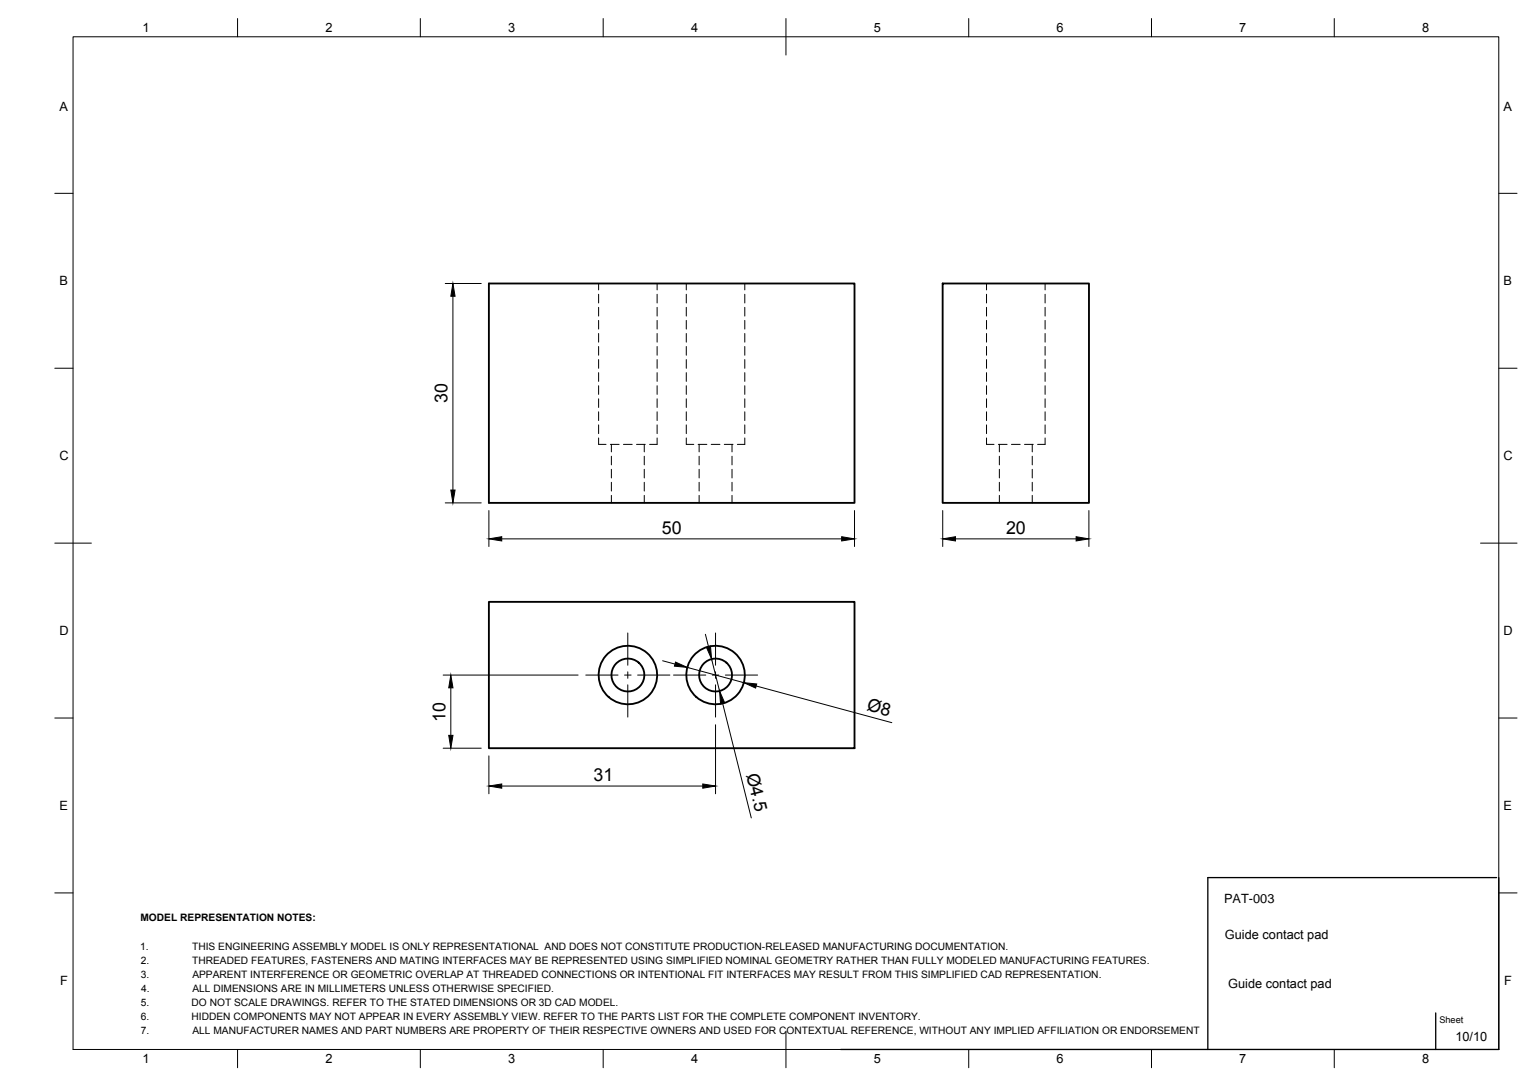
ISO-10303-21;
HEADER;
/* Generated by software containing ST-Developer
 * from STEP Tools, Inc. (www.steptools.com) 
 */

FILE_DESCRIPTION(
/* description */ ('PAT-003'),
/* implementation_level */ '2;1');

FILE_NAME(
/* name */ 'Guide contact pad.step',
/* time_stamp */ '2026-10-29T15:45:40-07:00',
/* author */ (''),
/* organization */ (''),
/* preprocessor_version */ 'ST-DEVELOPER v20.2',
/* originating_system */ 'Autodesk Translation Framework v15.17.0.0',
/* authorisation */ '');

FILE_SCHEMA (('AUTOMOTIVE_DESIGN { 1 0 10303 214 3 1 1 }'));
ENDSEC;

DATA;
#10=MECHANICAL_DESIGN_GEOMETRIC_PRESENTATION_REPRESENTATION('',(#154),#5761);
#130=SHAPE_REPRESENTATION_RELATIONSHIP('SRR','None',#5825,#142);
#142=ADVANCED_BREP_SHAPE_REPRESENTATION('',(#165),#5756);
#154=STYLED_ITEM('',(#5942),#165);
#165=MANIFOLD_SOLID_BREP('Body1',#3329);
#192=FACE_BOUND('',#674,.T.);
#193=FACE_BOUND('',#677,.T.);
#194=FACE_BOUND('',#685,.T.);
#195=FACE_BOUND('',#686,.T.);
#196=FACE_BOUND('',#688,.T.);
#197=FACE_BOUND('',#689,.T.);
#303=PLANE('',#3651);
#304=PLANE('',#3656);
#305=PLANE('',#3662);
#306=PLANE('',#3663);
#307=PLANE('',#3664);
#308=PLANE('',#3665);
#309=PLANE('',#3666);
#310=PLANE('',#3667);
#462=FACE_OUTER_BOUND('',#672,.T.);
#463=FACE_OUTER_BOUND('',#673,.T.);
#464=FACE_OUTER_BOUND('',#675,.T.);
#465=FACE_OUTER_BOUND('',#676,.T.);
#466=FACE_OUTER_BOUND('',#678,.T.);
#467=FACE_OUTER_BOUND('',#679,.T.);
#468=FACE_OUTER_BOUND('',#680,.T.);
#469=FACE_OUTER_BOUND('',#681,.T.);
#470=FACE_OUTER_BOUND('',#682,.T.);
#471=FACE_OUTER_BOUND('',#683,.T.);
#472=FACE_OUTER_BOUND('',#684,.T.);
#473=FACE_OUTER_BOUND('',#687,.T.);
#672=EDGE_LOOP('',(#2806,#2807,#2808,#2809));
#673=EDGE_LOOP('',(#2810));
#674=EDGE_LOOP('',(#2811));
#675=EDGE_LOOP('',(#2812,#2813,#2814,#2815));
#676=EDGE_LOOP('',(#2816));
#677=EDGE_LOOP('',(#2817));
#678=EDGE_LOOP('',(#2818,#2819,#2820,#2821));
#679=EDGE_LOOP('',(#2822,#2823,#2824,#2825));
#680=EDGE_LOOP('',(#2826,#2827,#2828,#2829));
#681=EDGE_LOOP('',(#2830,#2831,#2832,#2833));
#682=EDGE_LOOP('',(#2834,#2835,#2836,#2837));
#683=EDGE_LOOP('',(#2838,#2839,#2840,#2841));
#684=EDGE_LOOP('',(#2842,#2843,#2844,#2845));
#685=EDGE_LOOP('',(#2846));
#686=EDGE_LOOP('',(#2847));
#687=EDGE_LOOP('',(#2848,#2849,#2850,#2851));
#688=EDGE_LOOP('',(#2852));
#689=EDGE_LOOP('',(#2853));
#992=LINE('',#5383,#1314);
#993=LINE('',#5392,#1315);
#994=LINE('',#5400,#1316);
#995=LINE('',#5404,#1317);
#996=LINE('',#5408,#1318);
#997=LINE('',#5410,#1319);
#998=LINE('',#5412,#1320);
#999=LINE('',#5413,#1321);
#1000=LINE('',#5416,#1322);
#1001=LINE('',#5418,#1323);
#1002=LINE('',#5419,#1324);
#1003=LINE('',#5422,#1325);
#1004=LINE('',#5424,#1326);
#1005=LINE('',#5425,#1327);
#1006=LINE('',#5427,#1328);
#1007=LINE('',#5428,#1329);
#1314=VECTOR('',#4391,0.4);
#1315=VECTOR('',#4402,0.4);
#1316=VECTOR('',#4413,0.225);
#1317=VECTOR('',#4418,0.225);
#1318=VECTOR('',#4421,1.);
#1319=VECTOR('',#4422,1.);
#1320=VECTOR('',#4423,1.);
#1321=VECTOR('',#4424,1.);
#1322=VECTOR('',#4427,1.);
#1323=VECTOR('',#4428,1.);
#1324=VECTOR('',#4429,1.);
#1325=VECTOR('',#4432,1.);
#1326=VECTOR('',#4433,1.);
#1327=VECTOR('',#4434,1.);
#1328=VECTOR('',#4437,1.);
#1329=VECTOR('',#4438,1.);
#1442=CIRCLE('',#3649,0.4);
#1443=CIRCLE('',#3650,0.4);
#1444=CIRCLE('',#3652,0.225);
#1445=CIRCLE('',#3654,0.4);
#1446=CIRCLE('',#3655,0.4);
#1447=CIRCLE('',#3657,0.225);
#1448=CIRCLE('',#3659,0.225);
#1449=CIRCLE('',#3661,0.225);
#1686=VERTEX_POINT('',#5380);
#1687=VERTEX_POINT('',#5382);
#1688=VERTEX_POINT('',#5386);
#1689=VERTEX_POINT('',#5389);
#1690=VERTEX_POINT('',#5391);
#1691=VERTEX_POINT('',#5395);
#1692=VERTEX_POINT('',#5398);
#1693=VERTEX_POINT('',#5402);
#1694=VERTEX_POINT('',#5406);
#1695=VERTEX_POINT('',#5407);
#1696=VERTEX_POINT('',#5409);
#1697=VERTEX_POINT('',#5411);
#1698=VERTEX_POINT('',#5415);
#1699=VERTEX_POINT('',#5417);
#1700=VERTEX_POINT('',#5421);
#1701=VERTEX_POINT('',#5423);
#2074=EDGE_CURVE('',#1686,#1686,#1442,.T.);
#2075=EDGE_CURVE('',#1686,#1687,#992,.T.);
#2076=EDGE_CURVE('',#1687,#1687,#1443,.T.);
#2077=EDGE_CURVE('',#1688,#1688,#1444,.T.);
#2078=EDGE_CURVE('',#1689,#1689,#1445,.T.);
#2079=EDGE_CURVE('',#1689,#1690,#993,.T.);
#2080=EDGE_CURVE('',#1690,#1690,#1446,.T.);
#2081=EDGE_CURVE('',#1691,#1691,#1447,.T.);
#2082=EDGE_CURVE('',#1692,#1692,#1448,.T.);
#2083=EDGE_CURVE('',#1692,#1688,#994,.T.);
#2084=EDGE_CURVE('',#1693,#1693,#1449,.T.);
#2085=EDGE_CURVE('',#1693,#1691,#995,.T.);
#2086=EDGE_CURVE('',#1694,#1695,#996,.T.);
#2087=EDGE_CURVE('',#1695,#1696,#997,.T.);
#2088=EDGE_CURVE('',#1697,#1696,#998,.T.);
#2089=EDGE_CURVE('',#1694,#1697,#999,.T.);
#2090=EDGE_CURVE('',#1698,#1694,#1000,.T.);
#2091=EDGE_CURVE('',#1699,#1697,#1001,.T.);
#2092=EDGE_CURVE('',#1698,#1699,#1002,.T.);
#2093=EDGE_CURVE('',#1700,#1698,#1003,.T.);
#2094=EDGE_CURVE('',#1701,#1699,#1004,.T.);
#2095=EDGE_CURVE('',#1700,#1701,#1005,.T.);
#2096=EDGE_CURVE('',#1695,#1700,#1006,.T.);
#2097=EDGE_CURVE('',#1696,#1701,#1007,.T.);
#2806=ORIENTED_EDGE('',*,*,#2074,.F.);
#2807=ORIENTED_EDGE('',*,*,#2075,.T.);
#2808=ORIENTED_EDGE('',*,*,#2076,.F.);
#2809=ORIENTED_EDGE('',*,*,#2075,.F.);
#2810=ORIENTED_EDGE('',*,*,#2074,.T.);
#2811=ORIENTED_EDGE('',*,*,#2077,.F.);
#2812=ORIENTED_EDGE('',*,*,#2078,.F.);
#2813=ORIENTED_EDGE('',*,*,#2079,.T.);
#2814=ORIENTED_EDGE('',*,*,#2080,.F.);
#2815=ORIENTED_EDGE('',*,*,#2079,.F.);
#2816=ORIENTED_EDGE('',*,*,#2078,.T.);
#2817=ORIENTED_EDGE('',*,*,#2081,.F.);
#2818=ORIENTED_EDGE('',*,*,#2082,.F.);
#2819=ORIENTED_EDGE('',*,*,#2083,.T.);
#2820=ORIENTED_EDGE('',*,*,#2077,.T.);
#2821=ORIENTED_EDGE('',*,*,#2083,.F.);
#2822=ORIENTED_EDGE('',*,*,#2084,.F.);
#2823=ORIENTED_EDGE('',*,*,#2085,.T.);
#2824=ORIENTED_EDGE('',*,*,#2081,.T.);
#2825=ORIENTED_EDGE('',*,*,#2085,.F.);
#2826=ORIENTED_EDGE('',*,*,#2086,.T.);
#2827=ORIENTED_EDGE('',*,*,#2087,.T.);
#2828=ORIENTED_EDGE('',*,*,#2088,.F.);
#2829=ORIENTED_EDGE('',*,*,#2089,.F.);
#2830=ORIENTED_EDGE('',*,*,#2090,.T.);
#2831=ORIENTED_EDGE('',*,*,#2089,.T.);
#2832=ORIENTED_EDGE('',*,*,#2091,.F.);
#2833=ORIENTED_EDGE('',*,*,#2092,.F.);
#2834=ORIENTED_EDGE('',*,*,#2093,.T.);
#2835=ORIENTED_EDGE('',*,*,#2092,.T.);
#2836=ORIENTED_EDGE('',*,*,#2094,.F.);
#2837=ORIENTED_EDGE('',*,*,#2095,.F.);
#2838=ORIENTED_EDGE('',*,*,#2096,.T.);
#2839=ORIENTED_EDGE('',*,*,#2095,.T.);
#2840=ORIENTED_EDGE('',*,*,#2097,.F.);
#2841=ORIENTED_EDGE('',*,*,#2087,.F.);
#2842=ORIENTED_EDGE('',*,*,#2097,.T.);
#2843=ORIENTED_EDGE('',*,*,#2094,.T.);
#2844=ORIENTED_EDGE('',*,*,#2091,.T.);
#2845=ORIENTED_EDGE('',*,*,#2088,.T.);
#2846=ORIENTED_EDGE('',*,*,#2076,.T.);
#2847=ORIENTED_EDGE('',*,*,#2080,.T.);
#2848=ORIENTED_EDGE('',*,*,#2096,.F.);
#2849=ORIENTED_EDGE('',*,*,#2086,.F.);
#2850=ORIENTED_EDGE('',*,*,#2090,.F.);
#2851=ORIENTED_EDGE('',*,*,#2093,.F.);
#2852=ORIENTED_EDGE('',*,*,#2082,.T.);
#2853=ORIENTED_EDGE('',*,*,#2084,.T.);
#3112=CYLINDRICAL_SURFACE('',#3648,0.4);
#3113=CYLINDRICAL_SURFACE('',#3653,0.4);
#3114=CYLINDRICAL_SURFACE('',#3658,0.225);
#3115=CYLINDRICAL_SURFACE('',#3660,0.225);
#3255=ADVANCED_FACE('',(#462),#3112,.F.);
#3256=ADVANCED_FACE('',(#463,#192),#303,.T.);
#3257=ADVANCED_FACE('',(#464),#3113,.F.);
#3258=ADVANCED_FACE('',(#465,#193),#304,.T.);
#3259=ADVANCED_FACE('',(#466),#3114,.F.);
#3260=ADVANCED_FACE('',(#467),#3115,.F.);
#3261=ADVANCED_FACE('',(#468),#305,.T.);
#3262=ADVANCED_FACE('',(#469),#306,.T.);
#3263=ADVANCED_FACE('',(#470),#307,.T.);
#3264=ADVANCED_FACE('',(#471),#308,.T.);
#3265=ADVANCED_FACE('',(#472,#194,#195),#309,.T.);
#3266=ADVANCED_FACE('',(#473,#196,#197),#310,.F.);
#3329=CLOSED_SHELL('',(#3255,#3256,#3257,#3258,#3259,#3260,#3261,#3262,
#3263,#3264,#3265,#3266));
#3647=AXIS2_PLACEMENT_3D('',#5378,#4385,#4386);
#3648=AXIS2_PLACEMENT_3D('',#5379,#4387,#4388);
#3649=AXIS2_PLACEMENT_3D('',#5381,#4389,#4390);
#3650=AXIS2_PLACEMENT_3D('',#5384,#4392,#4393);
#3651=AXIS2_PLACEMENT_3D('',#5385,#4394,#4395);
#3652=AXIS2_PLACEMENT_3D('',#5387,#4396,#4397);
#3653=AXIS2_PLACEMENT_3D('',#5388,#4398,#4399);
#3654=AXIS2_PLACEMENT_3D('',#5390,#4400,#4401);
#3655=AXIS2_PLACEMENT_3D('',#5393,#4403,#4404);
#3656=AXIS2_PLACEMENT_3D('',#5394,#4405,#4406);
#3657=AXIS2_PLACEMENT_3D('',#5396,#4407,#4408);
#3658=AXIS2_PLACEMENT_3D('',#5397,#4409,#4410);
#3659=AXIS2_PLACEMENT_3D('',#5399,#4411,#4412);
#3660=AXIS2_PLACEMENT_3D('',#5401,#4414,#4415);
#3661=AXIS2_PLACEMENT_3D('',#5403,#4416,#4417);
#3662=AXIS2_PLACEMENT_3D('',#5405,#4419,#4420);
#3663=AXIS2_PLACEMENT_3D('',#5414,#4425,#4426);
#3664=AXIS2_PLACEMENT_3D('',#5420,#4430,#4431);
#3665=AXIS2_PLACEMENT_3D('',#5426,#4435,#4436);
#3666=AXIS2_PLACEMENT_3D('',#5429,#4439,#4440);
#3667=AXIS2_PLACEMENT_3D('',#5430,#4441,#4442);
#4385=DIRECTION('axis',(0.,0.,1.));
#4386=DIRECTION('refdir',(1.,0.,0.));
#4387=DIRECTION('center_axis',(0.,0.,1.));
#4388=DIRECTION('ref_axis',(1.,0.,0.));
#4389=DIRECTION('center_axis',(0.,0.,1.));
#4390=DIRECTION('ref_axis',(1.,0.,0.));
#4391=DIRECTION('',(0.,0.,1.));
#4392=DIRECTION('center_axis',(0.,0.,-1.));
#4393=DIRECTION('ref_axis',(1.,0.,0.));
#4394=DIRECTION('center_axis',(0.,0.,1.));
#4395=DIRECTION('ref_axis',(1.,0.,0.));
#4396=DIRECTION('center_axis',(0.,0.,1.));
#4397=DIRECTION('ref_axis',(1.,0.,0.));
#4398=DIRECTION('center_axis',(0.,0.,1.));
#4399=DIRECTION('ref_axis',(1.,0.,0.));
#4400=DIRECTION('center_axis',(0.,0.,1.));
#4401=DIRECTION('ref_axis',(1.,0.,0.));
#4402=DIRECTION('',(0.,0.,1.));
#4403=DIRECTION('center_axis',(0.,0.,-1.));
#4404=DIRECTION('ref_axis',(1.,0.,0.));
#4405=DIRECTION('center_axis',(0.,0.,1.));
#4406=DIRECTION('ref_axis',(1.,0.,0.));
#4407=DIRECTION('center_axis',(0.,0.,1.));
#4408=DIRECTION('ref_axis',(1.,0.,0.));
#4409=DIRECTION('center_axis',(0.,0.,1.));
#4410=DIRECTION('ref_axis',(1.,0.,0.));
#4411=DIRECTION('center_axis',(0.,0.,1.));
#4412=DIRECTION('ref_axis',(1.,0.,0.));
#4413=DIRECTION('',(0.,0.,1.));
#4414=DIRECTION('center_axis',(0.,0.,1.));
#4415=DIRECTION('ref_axis',(1.,0.,0.));
#4416=DIRECTION('center_axis',(0.,0.,1.));
#4417=DIRECTION('ref_axis',(1.,0.,0.));
#4418=DIRECTION('',(0.,0.,1.));
#4419=DIRECTION('center_axis',(0.,1.,0.));
#4420=DIRECTION('ref_axis',(-1.,0.,0.));
#4421=DIRECTION('',(-1.,0.,0.));
#4422=DIRECTION('',(0.,0.,1.));
#4423=DIRECTION('',(-1.,0.,0.));
#4424=DIRECTION('',(0.,0.,1.));
#4425=DIRECTION('center_axis',(1.,0.,0.));
#4426=DIRECTION('ref_axis',(0.,1.,0.));
#4427=DIRECTION('',(0.,1.,0.));
#4428=DIRECTION('',(0.,1.,0.));
#4429=DIRECTION('',(0.,0.,1.));
#4430=DIRECTION('center_axis',(0.,-1.,0.));
#4431=DIRECTION('ref_axis',(1.,0.,0.));
#4432=DIRECTION('',(1.,0.,0.));
#4433=DIRECTION('',(1.,0.,0.));
#4434=DIRECTION('',(0.,0.,1.));
#4435=DIRECTION('center_axis',(-1.,0.,0.));
#4436=DIRECTION('ref_axis',(0.,-1.,0.));
#4437=DIRECTION('',(0.,-1.,0.));
#4438=DIRECTION('',(0.,-1.,0.));
#4439=DIRECTION('center_axis',(0.,0.,1.));
#4440=DIRECTION('ref_axis',(1.,0.,0.));
#4441=DIRECTION('center_axis',(0.,0.,1.));
#4442=DIRECTION('ref_axis',(1.,0.,0.));
#5378=CARTESIAN_POINT('',(0.,0.,0.));
#5379=CARTESIAN_POINT('Origin',(14.,-0.6,6.4));
#5380=CARTESIAN_POINT('',(13.6,-0.6,6.4));
#5381=CARTESIAN_POINT('Origin',(14.,-0.6,6.4));
#5382=CARTESIAN_POINT('',(13.6,-0.6,8.6));
#5383=CARTESIAN_POINT('',(13.6,-0.6,6.4));
#5384=CARTESIAN_POINT('Origin',(14.,-0.6,8.6));
#5385=CARTESIAN_POINT('Origin',(14.,-0.6,6.4));
#5386=CARTESIAN_POINT('',(13.775,-0.6,6.4));
#5387=CARTESIAN_POINT('Origin',(14.,-0.6,6.4));
#5388=CARTESIAN_POINT('Origin',(14.,0.6,6.4));
#5389=CARTESIAN_POINT('',(13.6,0.6,6.4));
#5390=CARTESIAN_POINT('Origin',(14.,0.6,6.4));
#5391=CARTESIAN_POINT('',(13.6,0.6,8.6));
#5392=CARTESIAN_POINT('',(13.6,0.6,6.4));
#5393=CARTESIAN_POINT('Origin',(14.,0.6,8.6));
#5394=CARTESIAN_POINT('Origin',(14.,0.6,6.4));
#5395=CARTESIAN_POINT('',(13.775,0.6,6.4));
#5396=CARTESIAN_POINT('Origin',(14.,0.6,6.4));
#5397=CARTESIAN_POINT('Origin',(14.,-0.6,5.5));
#5398=CARTESIAN_POINT('',(13.775,-0.6,5.6));
#5399=CARTESIAN_POINT('Origin',(14.,-0.6,5.6));
#5400=CARTESIAN_POINT('',(13.775,-0.6,5.5));
#5401=CARTESIAN_POINT('Origin',(14.,0.6,5.5));
#5402=CARTESIAN_POINT('',(13.775,0.6,5.6));
#5403=CARTESIAN_POINT('Origin',(14.,0.6,5.6));
#5404=CARTESIAN_POINT('',(13.775,0.6,5.5));
#5405=CARTESIAN_POINT('Origin',(15.,2.5,5.6));
#5406=CARTESIAN_POINT('',(15.,2.5,5.6));
#5407=CARTESIAN_POINT('',(13.,2.5,5.6));
#5408=CARTESIAN_POINT('',(15.,2.5,5.6));
#5409=CARTESIAN_POINT('',(13.,2.5,8.6));
#5410=CARTESIAN_POINT('',(13.,2.5,5.6));
#5411=CARTESIAN_POINT('',(15.,2.5,8.6));
#5412=CARTESIAN_POINT('',(15.,2.5,8.6));
#5413=CARTESIAN_POINT('',(15.,2.5,5.6));
#5414=CARTESIAN_POINT('Origin',(15.,-2.5,5.6));
#5415=CARTESIAN_POINT('',(15.,-2.5,5.6));
#5416=CARTESIAN_POINT('',(15.,-2.5,5.6));
#5417=CARTESIAN_POINT('',(15.,-2.5,8.6));
#5418=CARTESIAN_POINT('',(15.,-2.5,8.6));
#5419=CARTESIAN_POINT('',(15.,-2.5,5.6));
#5420=CARTESIAN_POINT('Origin',(13.,-2.5,5.6));
#5421=CARTESIAN_POINT('',(13.,-2.5,5.6));
#5422=CARTESIAN_POINT('',(13.,-2.5,5.6));
#5423=CARTESIAN_POINT('',(13.,-2.5,8.6));
#5424=CARTESIAN_POINT('',(13.,-2.5,8.6));
#5425=CARTESIAN_POINT('',(13.,-2.5,5.6));
#5426=CARTESIAN_POINT('Origin',(13.,2.5,5.6));
#5427=CARTESIAN_POINT('',(13.,2.5,5.6));
#5428=CARTESIAN_POINT('',(13.,2.5,8.6));
#5429=CARTESIAN_POINT('Origin',(14.,0.,8.6));
#5430=CARTESIAN_POINT('Origin',(14.,0.,5.6));
#5740=UNCERTAINTY_MEASURE_WITH_UNIT(LENGTH_MEASURE(0.001),#5762,
'DISTANCE_ACCURACY_VALUE',
'Maximum model space distance between geometric entities at asserted c
onnectivities');
#5745=UNCERTAINTY_MEASURE_WITH_UNIT(LENGTH_MEASURE(0.001),#5762,
'DISTANCE_ACCURACY_VALUE',
'Maximum model space distance between geometric entities at asserted c
onnectivities');
#5756=(
GEOMETRIC_REPRESENTATION_CONTEXT(3)
GLOBAL_UNCERTAINTY_ASSIGNED_CONTEXT((#5740))
GLOBAL_UNIT_ASSIGNED_CONTEXT((#5762,#5764,#5765))
REPRESENTATION_CONTEXT('','3D')
);
#5761=(
GEOMETRIC_REPRESENTATION_CONTEXT(3)
GLOBAL_UNCERTAINTY_ASSIGNED_CONTEXT((#5745))
GLOBAL_UNIT_ASSIGNED_CONTEXT((#5762,#5764,#5765))
REPRESENTATION_CONTEXT('','3D')
);
#5762=(
LENGTH_UNIT()
NAMED_UNIT(*)
SI_UNIT(.CENTI.,.METRE.)
);
#5764=(
NAMED_UNIT(*)
PLANE_ANGLE_UNIT()
SI_UNIT($,.RADIAN.)
);
#5765=(
NAMED_UNIT(*)
SI_UNIT($,.STERADIAN.)
SOLID_ANGLE_UNIT()
);
#5776=SHAPE_DEFINITION_REPRESENTATION(#5791,#5825);
#5791=PRODUCT_DEFINITION_SHAPE('',$,#5841);
#5825=SHAPE_REPRESENTATION('',(#3647),#5756);
#5830=PRODUCT_DEFINITION_CONTEXT('part definition',#5877,'design');
#5841=PRODUCT_DEFINITION('Guide contact pad','Guide contact pad',#5856,
#5830);
#5856=PRODUCT_DEFINITION_FORMATION('',$,#5889);
#5877=APPLICATION_CONTEXT(
'Core Data for Automotive Mechanical Design Process');
#5878=PRODUCT_CONTEXT('part definition',#5877,'mechanical');
#5889=PRODUCT('Guide contact pad','Guide contact pad',
'Guide contact pad',(#5878));
#5936=COLOUR_RGB('Sky Blue',0.24,0.69,0.87);
#5937=FILL_AREA_STYLE_COLOUR('',#5936);
#5938=FILL_AREA_STYLE('',(#5937));
#5939=SURFACE_STYLE_FILL_AREA(#5938);
#5940=SURFACE_SIDE_STYLE('',(#5939));
#5941=SURFACE_STYLE_USAGE(.BOTH.,#5940);
#5942=PRESENTATION_STYLE_ASSIGNMENT((#5941));
ENDSEC;
END-ISO-10303-21;
